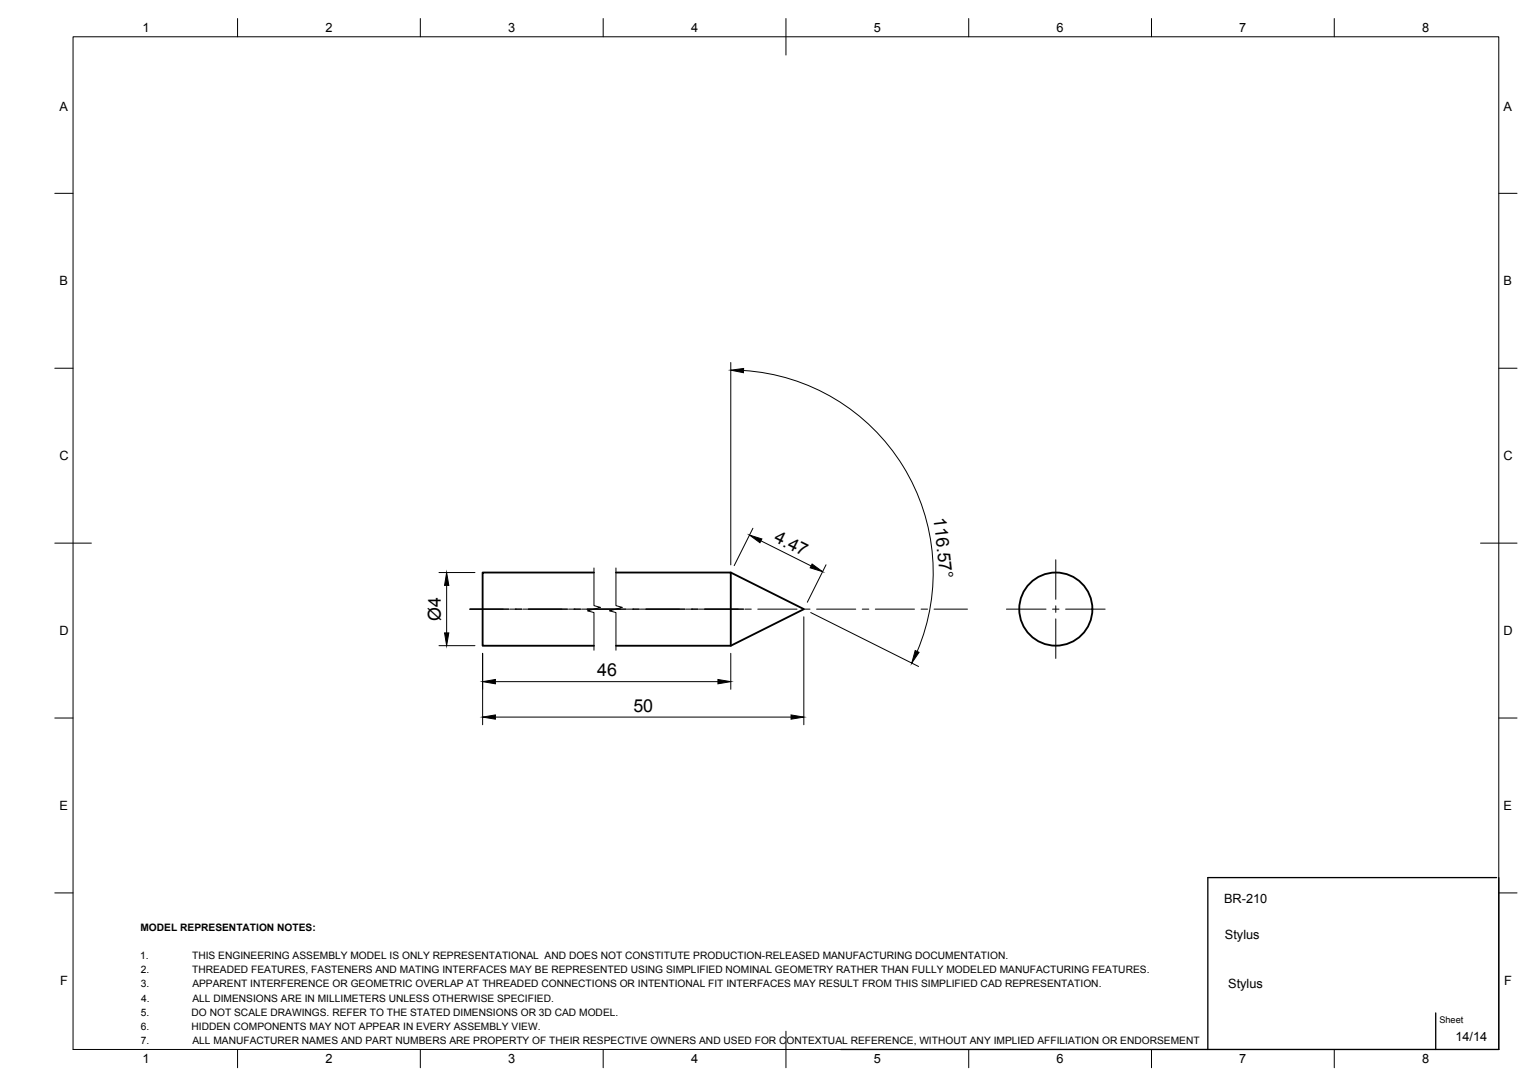
ISO-10303-21;
HEADER;
/* Generated by software containing ST-Developer
 * from STEP Tools, Inc. (www.steptools.com) 
 */

FILE_DESCRIPTION(
/* description */ ('Independent 1:2 reduction pantograph. 120 mm parallelogram sides; fix
ed fulcrum on the extension of a 240 mm link. Drawing point halfway al
ong its link, so its XY displacement is one half of the tracing point.
 Replaceable pivot bushes and retained pins. Calibration and productio
n accuracy unassigned.'),
/* implementation_level */ '2;1');

FILE_NAME(
/* name */ 'Stylus.step',
/* time_stamp */ '2026-11-07T22:11:57-08:00',
/* author */ (''),
/* organization */ (''),
/* preprocessor_version */ 'ST-DEVELOPER v20.2',
/* originating_system */ 'Autodesk Translation Framework v15.17.0.0',
/* authorisation */ '');

FILE_SCHEMA (('AUTOMOTIVE_DESIGN { 1 0 10303 214 3 1 1 }'));
ENDSEC;

DATA;
#10=MECHANICAL_DESIGN_GEOMETRIC_PRESENTATION_REPRESENTATION('',(#198),#2926);
#159=CONICAL_SURFACE('',#1891,1.,0.463647609000806);
#172=SHAPE_REPRESENTATION_RELATIONSHIP('SRR','None',#3009,#185);
#185=ADVANCED_BREP_SHAPE_REPRESENTATION('',(#211),#2925);
#198=STYLED_ITEM('',(#3081),#211);
#211=MANIFOLD_SOLID_BREP('Body1',#1553);
#304=PLANE('',#1890);
#394=FACE_OUTER_BOUND('',#532,.T.);
#395=FACE_OUTER_BOUND('',#533,.T.);
#396=FACE_OUTER_BOUND('',#534,.T.);
#532=EDGE_LOOP('',(#1397,#1398,#1399,#1400));
#533=EDGE_LOOP('',(#1401));
#534=EDGE_LOOP('',(#1402,#1403,#1404));
#614=LINE('',#2854,#695);
#615=LINE('',#2859,#696);
#695=VECTOR('',#2390,2.);
#696=VECTOR('',#2397,1.);
#783=CIRCLE('',#1888,2.);
#784=CIRCLE('',#1889,2.);
#895=VERTEX_POINT('',#2851);
#896=VERTEX_POINT('',#2853);
#897=VERTEX_POINT('',#2858);
#1063=EDGE_CURVE('',#895,#895,#783,.T.);
#1064=EDGE_CURVE('',#895,#896,#614,.T.);
#1065=EDGE_CURVE('',#896,#896,#784,.T.);
#1066=EDGE_CURVE('',#896,#897,#615,.T.);
#1397=ORIENTED_EDGE('',*,*,#1063,.F.);
#1398=ORIENTED_EDGE('',*,*,#1064,.T.);
#1399=ORIENTED_EDGE('',*,*,#1065,.T.);
#1400=ORIENTED_EDGE('',*,*,#1064,.F.);
#1401=ORIENTED_EDGE('',*,*,#1063,.T.);
#1402=ORIENTED_EDGE('',*,*,#1065,.F.);
#1403=ORIENTED_EDGE('',*,*,#1066,.T.);
#1404=ORIENTED_EDGE('',*,*,#1066,.F.);
#1448=CYLINDRICAL_SURFACE('',#1887,2.);
#1538=ADVANCED_FACE('',(#394),#1448,.T.);
#1539=ADVANCED_FACE('',(#395),#304,.T.);
#1540=ADVANCED_FACE('',(#396),#159,.T.);
#1553=CLOSED_SHELL('',(#1538,#1539,#1540));
#1886=AXIS2_PLACEMENT_3D('',#2849,#2384,#2385);
#1887=AXIS2_PLACEMENT_3D('',#2850,#2386,#2387);
#1888=AXIS2_PLACEMENT_3D('',#2852,#2388,#2389);
#1889=AXIS2_PLACEMENT_3D('',#2855,#2391,#2392);
#1890=AXIS2_PLACEMENT_3D('',#2856,#2393,#2394);
#1891=AXIS2_PLACEMENT_3D('',#2857,#2395,#2396);
#2384=DIRECTION('axis',(0.,0.,1.));
#2385=DIRECTION('refdir',(1.,0.,0.));
#2386=DIRECTION('center_axis',(0.,0.,1.));
#2387=DIRECTION('ref_axis',(1.,0.,0.));
#2388=DIRECTION('center_axis',(0.,0.,1.));
#2389=DIRECTION('ref_axis',(1.,0.,0.));
#2390=DIRECTION('',(0.,0.,-1.));
#2391=DIRECTION('center_axis',(0.,0.,1.));
#2392=DIRECTION('ref_axis',(1.,0.,0.));
#2393=DIRECTION('center_axis',(0.,0.,1.));
#2394=DIRECTION('ref_axis',(1.,0.,0.));
#2395=DIRECTION('center_axis',(0.,0.,1.));
#2396=DIRECTION('ref_axis',(1.,0.,0.));
#2397=DIRECTION('',(0.447213595499958,5.47678698264203E-17,-0.894427190999916));
#2849=CARTESIAN_POINT('',(0.,0.,0.));
#2850=CARTESIAN_POINT('Origin',(0.,0.,4.));
#2851=CARTESIAN_POINT('',(-2.,-2.44929359829471E-16,50.));
#2852=CARTESIAN_POINT('Origin',(0.,0.,50.));
#2853=CARTESIAN_POINT('',(-2.,-2.44929359829471E-16,4.));
#2854=CARTESIAN_POINT('',(-2.,-2.44929359829471E-16,4.));
#2855=CARTESIAN_POINT('Origin',(0.,0.,4.));
#2856=CARTESIAN_POINT('Origin',(0.,0.,50.));
#2857=CARTESIAN_POINT('Origin',(0.,0.,2.));
#2858=CARTESIAN_POINT('',(0.,0.,0.));
#2859=CARTESIAN_POINT('',(-1.,-1.22464679914735E-16,2.));
#2910=UNCERTAINTY_MEASURE_WITH_UNIT(LENGTH_MEASURE(0.01),#2927,
'DISTANCE_ACCURACY_VALUE',
'Maximum model space distance between geometric entities at asserted c
onnectivities');
#2911=UNCERTAINTY_MEASURE_WITH_UNIT(LENGTH_MEASURE(0.01),#2927,
'DISTANCE_ACCURACY_VALUE',
'Maximum model space distance between geometric entities at asserted c
onnectivities');
#2925=(
GEOMETRIC_REPRESENTATION_CONTEXT(3)
GLOBAL_UNCERTAINTY_ASSIGNED_CONTEXT((#2910))
GLOBAL_UNIT_ASSIGNED_CONTEXT((#2927,#2929,#2930))
REPRESENTATION_CONTEXT('','3D')
);
#2926=(
GEOMETRIC_REPRESENTATION_CONTEXT(3)
GLOBAL_UNCERTAINTY_ASSIGNED_CONTEXT((#2911))
GLOBAL_UNIT_ASSIGNED_CONTEXT((#2927,#2929,#2930))
REPRESENTATION_CONTEXT('','3D')
);
#2927=(
LENGTH_UNIT()
NAMED_UNIT(*)
SI_UNIT(.MILLI.,.METRE.)
);
#2929=(
NAMED_UNIT(*)
PLANE_ANGLE_UNIT()
SI_UNIT($,.RADIAN.)
);
#2930=(
NAMED_UNIT(*)
SI_UNIT($,.STERADIAN.)
SOLID_ANGLE_UNIT()
);
#2944=SHAPE_DEFINITION_REPRESENTATION(#2958,#3009);
#2958=PRODUCT_DEFINITION_SHAPE('',$,#3024);
#3009=SHAPE_REPRESENTATION('',(#1886),#2925);
#3010=PRODUCT_DEFINITION_CONTEXT('part definition',#3054,'design');
#3024=PRODUCT_DEFINITION('Stylus','Stylus',#3038,#3010);
#3038=PRODUCT_DEFINITION_FORMATION('',$,#3069);
#3054=APPLICATION_CONTEXT(
'Core Data for Automotive Mechanical Design Process');
#3055=PRODUCT_CONTEXT('part definition',#3054,'mechanical');
#3069=PRODUCT('Stylus','Stylus',$,(#3055));
#3081=PRESENTATION_STYLE_ASSIGNMENT((#3093));
#3093=SURFACE_STYLE_USAGE(.BOTH.,#3105);
#3105=SURFACE_SIDE_STYLE('',(#3117));
#3117=SURFACE_STYLE_FILL_AREA(#3129);
#3129=FILL_AREA_STYLE('Stylus light gray',(#3141));
#3141=FILL_AREA_STYLE_COLOUR('Stylus light gray',#3153);
#3153=COLOUR_RGB('Stylus light gray',0.725490196078431,0.752941176470588,
0.792156862745098);
ENDSEC;
END-ISO-10303-21;
